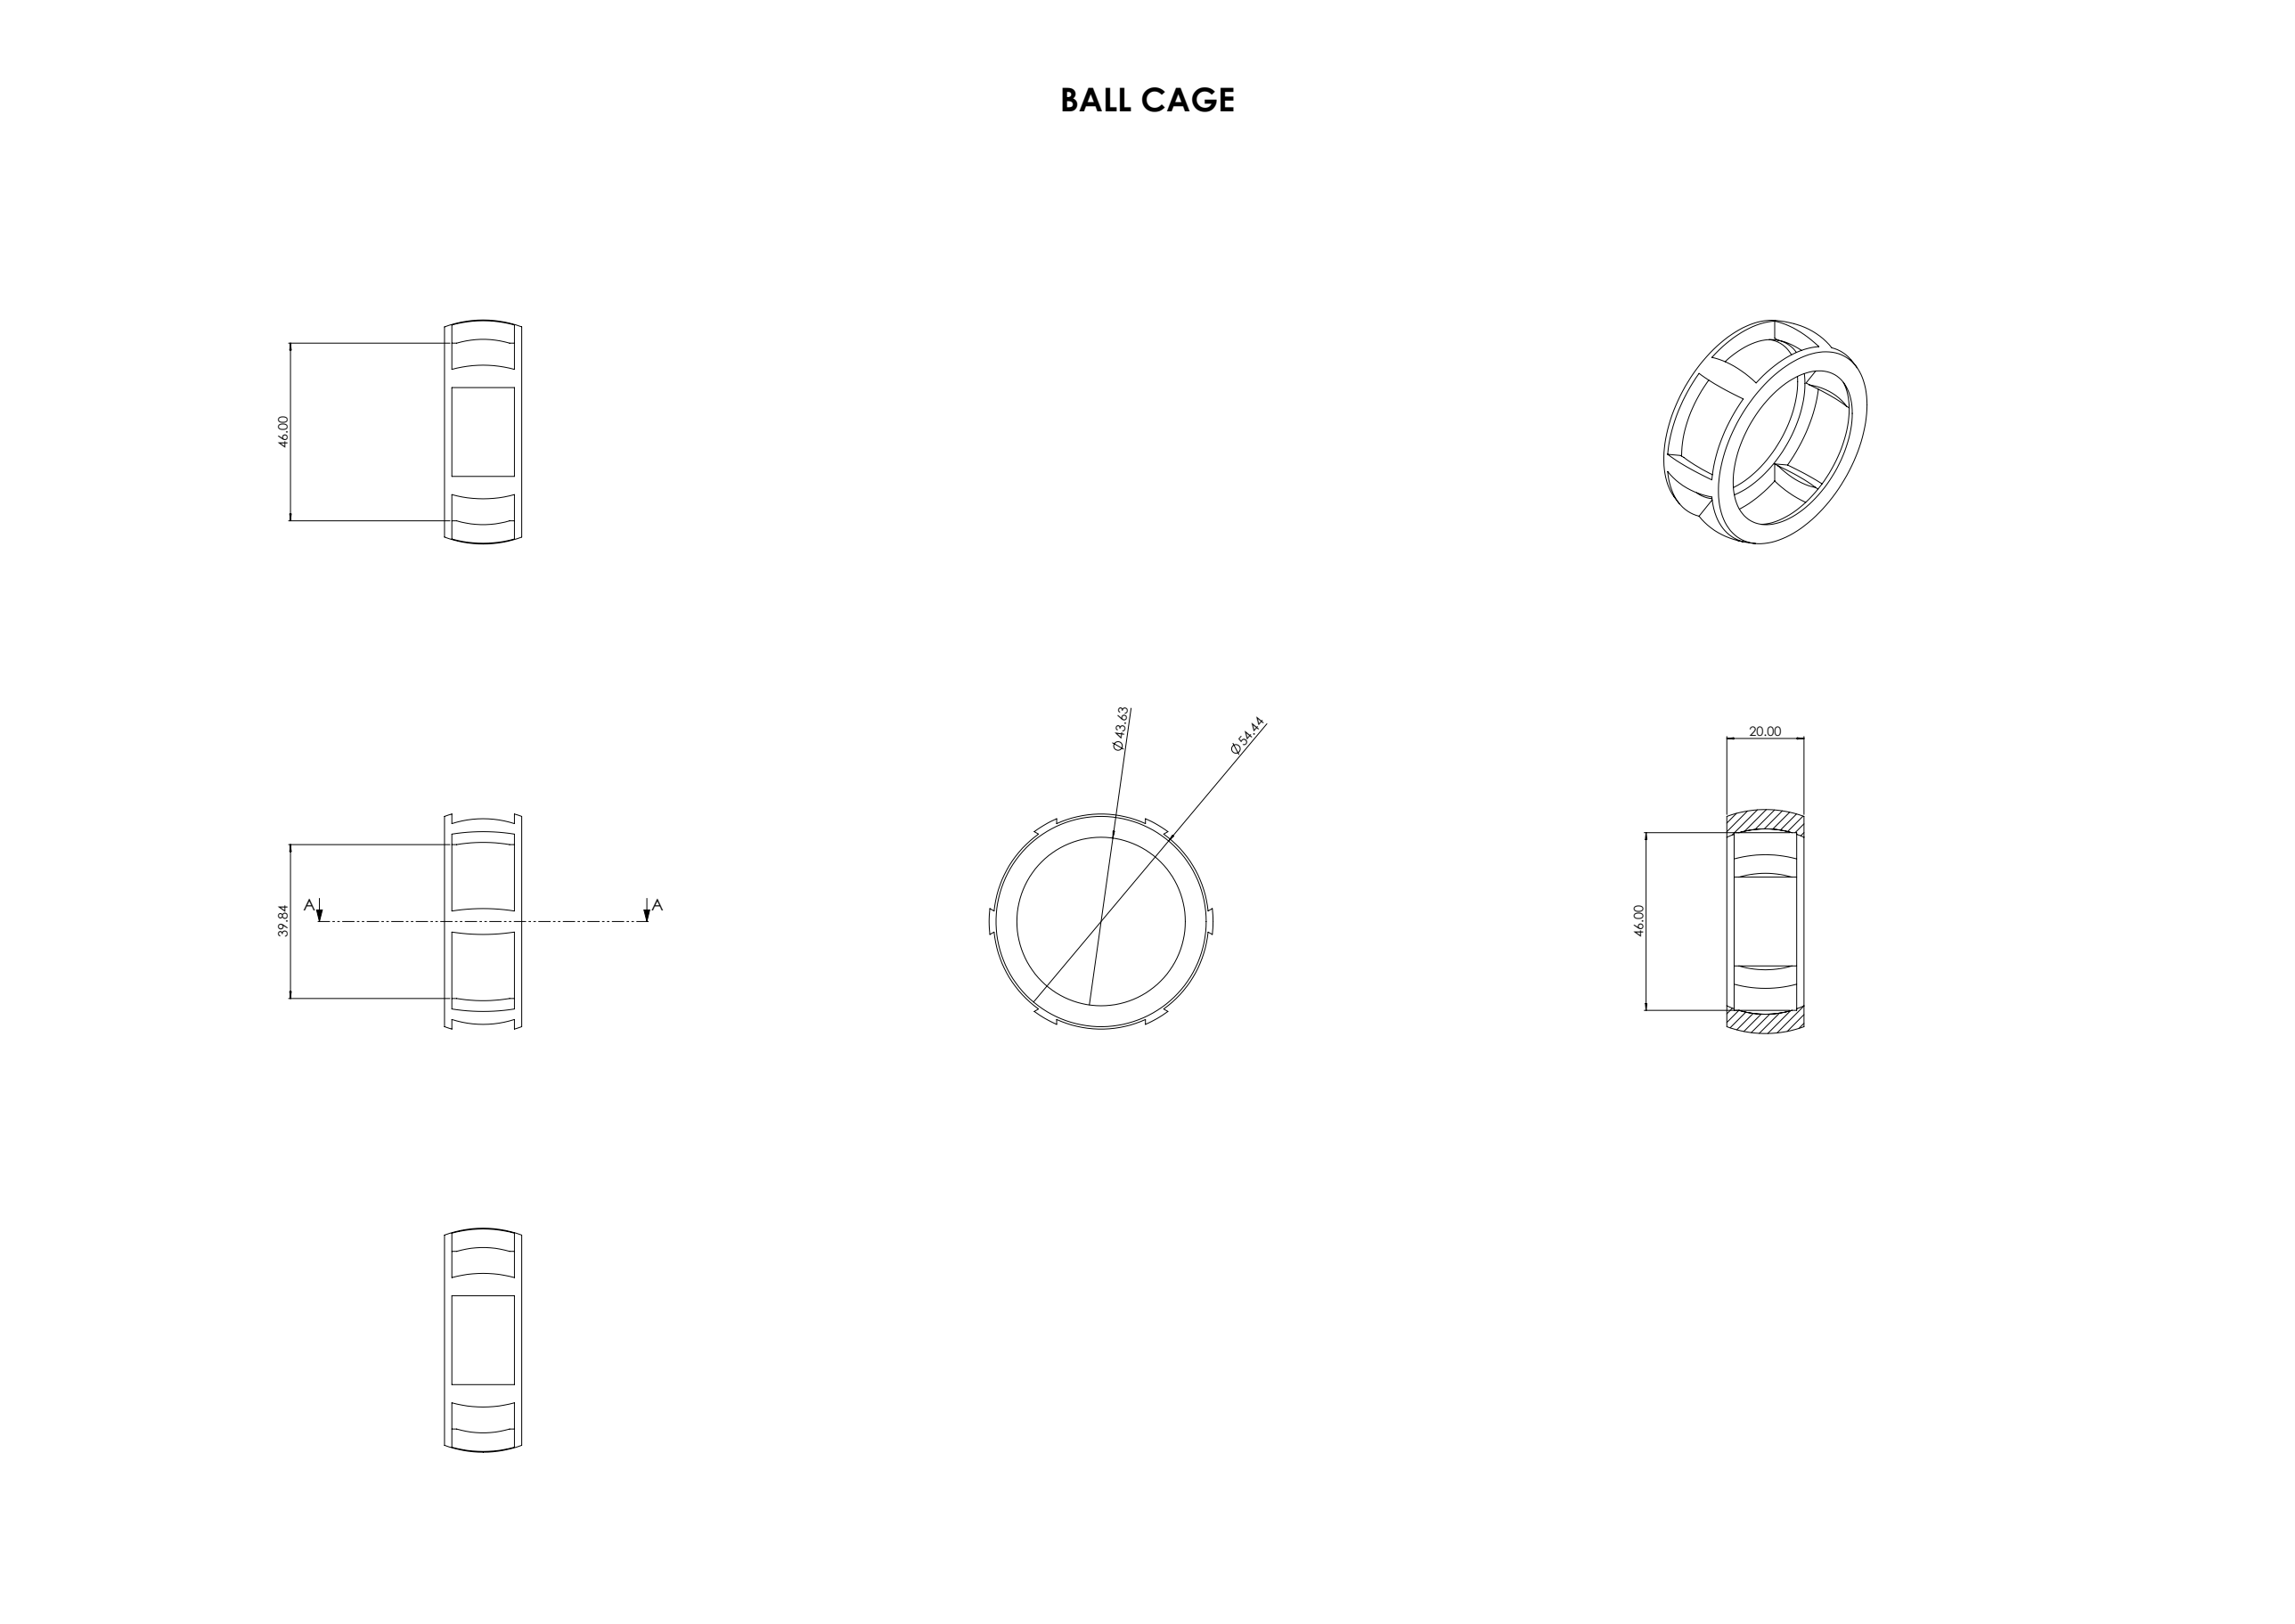
ISO-10303-21;
HEADER;
/* Generated by software containing ST-Developer
 * from STEP Tools, Inc. (www.steptools.com) 
 */

FILE_DESCRIPTION(
/* description */ (''),
/* implementation_level */ '2;1');

FILE_NAME(
/* name */ '05_Ball_Cage.step',
/* time_stamp */ '2026-10-11T12:57:03-07:00',
/* author */ (''),
/* organization */ (''),
/* preprocessor_version */ 'ST-DEVELOPER v20.2',
/* originating_system */ 'Autodesk Translation Framework v15.15.0.0',
/* authorisation */ '');

FILE_SCHEMA (('AUTOMOTIVE_DESIGN { 1 0 10303 214 3 1 1 }'));
ENDSEC;

DATA;
#10=MECHANICAL_DESIGN_GEOMETRIC_PRESENTATION_REPRESENTATION('',(#260),#90374);
#226=SHAPE_REPRESENTATION_RELATIONSHIP('SRR','None',#90445,#243);
#243=ADVANCED_BREP_SHAPE_REPRESENTATION('',(#277),#90361);
#260=STYLED_ITEM('',(#90701),#277);
#277=MANIFOLD_SOLID_BREP('Body1',#40349);
#557=SPHERICAL_SURFACE('',#43737,24.);
#558=SPHERICAL_SURFACE('',#43740,24.);
#559=SPHERICAL_SURFACE('',#43742,24.);
#560=SPHERICAL_SURFACE('',#43747,24.);
#561=SPHERICAL_SURFACE('',#43754,24.);
#562=SPHERICAL_SURFACE('',#43761,24.);
#563=SPHERICAL_SURFACE('',#43769,24.);
#564=SPHERICAL_SURFACE('',#43785,24.);
#565=SPHERICAL_SURFACE('',#43789,29.);
#1053=FACE_BOUND('',#6193,.T.);
#1054=FACE_BOUND('',#6196,.T.);
#1055=FACE_BOUND('',#6213,.T.);
#1056=FACE_BOUND('',#6215,.T.);
#1057=FACE_BOUND('',#6217,.T.);
#1058=FACE_BOUND('',#6219,.T.);
#1059=FACE_BOUND('',#6221,.T.);
#1060=FACE_BOUND('',#6222,.T.);
#1061=FACE_BOUND('',#6223,.T.);
#1062=FACE_BOUND('',#6224,.T.);
#1063=FACE_BOUND('',#6225,.T.);
#1064=FACE_BOUND('',#6226,.T.);
#1065=FACE_BOUND('',#6227,.T.);
#1420=PLANE('',#43720);
#1421=PLANE('',#43723);
#1422=PLANE('',#43726);
#1423=PLANE('',#43734);
#1424=PLANE('',#43744);
#1425=PLANE('',#43749);
#1426=PLANE('',#43751);
#1427=PLANE('',#43756);
#1428=PLANE('',#43758);
#1429=PLANE('',#43764);
#1430=PLANE('',#43766);
#1431=PLANE('',#43771);
#1432=PLANE('',#43773);
#1433=PLANE('',#43775);
#1434=PLANE('',#43782);
#1435=PLANE('',#43786);
#3780=FACE_OUTER_BOUND('',#6190,.T.);
#3781=FACE_OUTER_BOUND('',#6191,.T.);
#3782=FACE_OUTER_BOUND('',#6192,.T.);
#3783=FACE_OUTER_BOUND('',#6194,.T.);
#3784=FACE_OUTER_BOUND('',#6195,.T.);
#3785=FACE_OUTER_BOUND('',#6197,.T.);
#3786=FACE_OUTER_BOUND('',#6198,.T.);
#3787=FACE_OUTER_BOUND('',#6199,.T.);
#3788=FACE_OUTER_BOUND('',#6200,.T.);
#3789=FACE_OUTER_BOUND('',#6201,.T.);
#3790=FACE_OUTER_BOUND('',#6202,.T.);
#3791=FACE_OUTER_BOUND('',#6203,.T.);
#3792=FACE_OUTER_BOUND('',#6204,.T.);
#3793=FACE_OUTER_BOUND('',#6205,.T.);
#3794=FACE_OUTER_BOUND('',#6206,.T.);
#3795=FACE_OUTER_BOUND('',#6207,.T.);
#3796=FACE_OUTER_BOUND('',#6208,.T.);
#3797=FACE_OUTER_BOUND('',#6209,.T.);
#3798=FACE_OUTER_BOUND('',#6210,.T.);
#3799=FACE_OUTER_BOUND('',#6211,.T.);
#3800=FACE_OUTER_BOUND('',#6212,.T.);
#3801=FACE_OUTER_BOUND('',#6214,.T.);
#3802=FACE_OUTER_BOUND('',#6216,.T.);
#3803=FACE_OUTER_BOUND('',#6218,.T.);
#3804=FACE_OUTER_BOUND('',#6220,.T.);
#6190=EDGE_LOOP('',(#33099,#33100,#33101,#33102,#33103,#33104));
#6191=EDGE_LOOP('',(#33105,#33106,#33107,#33108,#33109,#33110));
#6192=EDGE_LOOP('',(#33111,#33112,#33113,#33114,#33115,#33116,#33117,#33118,
#33119,#33120,#33121,#33122,#33123,#33124,#33125,#33126,#33127,#33128));
#6193=EDGE_LOOP('',(#33129));
#6194=EDGE_LOOP('',(#33130,#33131,#33132,#33133,#33134,#33135));
#6195=EDGE_LOOP('',(#33136));
#6196=EDGE_LOOP('',(#33137));
#6197=EDGE_LOOP('',(#33138,#33139,#33140,#33141));
#6198=EDGE_LOOP('',(#33142,#33143));
#6199=EDGE_LOOP('',(#33144,#33145,#33146,#33147,#33148,#33149));
#6200=EDGE_LOOP('',(#33150,#33151));
#6201=EDGE_LOOP('',(#33152,#33153,#33154,#33155,#33156,#33157));
#6202=EDGE_LOOP('',(#33158,#33159,#33160,#33161,#33162,#33163));
#6203=EDGE_LOOP('',(#33164,#33165));
#6204=EDGE_LOOP('',(#33166,#33167,#33168,#33169,#33170,#33171));
#6205=EDGE_LOOP('',(#33172,#33173,#33174,#33175,#33176,#33177));
#6206=EDGE_LOOP('',(#33178,#33179,#33180,#33181));
#6207=EDGE_LOOP('',(#33182,#33183,#33184,#33185,#33186,#33187));
#6208=EDGE_LOOP('',(#33188,#33189,#33190,#33191,#33192,#33193));
#6209=EDGE_LOOP('',(#33194,#33195));
#6210=EDGE_LOOP('',(#33196,#33197,#33198,#33199,#33200,#33201));
#6211=EDGE_LOOP('',(#33202,#33203,#33204,#33205,#33206,#33207));
#6212=EDGE_LOOP('',(#33208,#33209,#33210,#33211,#33212,#33213,#33214,#33215,
#33216,#33217,#33218,#33219,#33220,#33221,#33222,#33223,#33224,#33225));
#6213=EDGE_LOOP('',(#33226));
#6214=EDGE_LOOP('',(#33227));
#6215=EDGE_LOOP('',(#33228));
#6216=EDGE_LOOP('',(#33229));
#6217=EDGE_LOOP('',(#33230));
#6218=EDGE_LOOP('',(#33231,#33232));
#6219=EDGE_LOOP('',(#33233));
#6220=EDGE_LOOP('',(#33234,#33235,#33236,#33237,#33238,#33239));
#6221=EDGE_LOOP('',(#33240,#33241,#33242,#33243));
#6222=EDGE_LOOP('',(#33244,#33245,#33246,#33247));
#6223=EDGE_LOOP('',(#33248,#33249,#33250,#33251));
#6224=EDGE_LOOP('',(#33252,#33253,#33254,#33255));
#6225=EDGE_LOOP('',(#33256,#33257,#33258,#33259));
#6226=EDGE_LOOP('',(#33260,#33261,#33262,#33263));
#6227=EDGE_LOOP('',(#33264));
#8631=CIRCLE('',#43721,26.6223590239483);
#8632=CIRCLE('',#43722,21.0653744329409);
#8633=CIRCLE('',#43724,26.6223590239483);
#8634=CIRCLE('',#43725,21.0653744329409);
#8635=CIRCLE('',#43727,27.8458255399261);
#8636=CIRCLE('',#43728,27.8458255399261);
#8637=CIRCLE('',#43729,27.8458255399261);
#8638=CIRCLE('',#43730,27.8458255399261);
#8639=CIRCLE('',#43731,27.8458255399261);
#8640=CIRCLE('',#43732,27.8458255399261);
#8641=CIRCLE('',#43733,22.5918126762773);
#8642=CIRCLE('',#43735,21.0653744329409);
#8643=CIRCLE('',#43736,26.6223590239483);
#8644=CIRCLE('',#43738,22.5918126762773);
#8645=CIRCLE('',#43739,21.8174242292714);
#8646=CIRCLE('',#43741,24.);
#8647=CIRCLE('',#43743,21.0653744329409);
#8648=CIRCLE('',#43745,26.6223590239483);
#8649=CIRCLE('',#43746,21.0653744329409);
#8650=CIRCLE('',#43748,21.0653744329409);
#8651=CIRCLE('',#43750,26.6223590239483);
#8652=CIRCLE('',#43752,26.6223590239483);
#8653=CIRCLE('',#43753,21.0653744329409);
#8654=CIRCLE('',#43755,21.0653744329409);
#8655=CIRCLE('',#43757,26.6223590239483);
#8656=CIRCLE('',#43759,26.6223590239483);
#8657=CIRCLE('',#43760,21.0653744329409);
#8658=CIRCLE('',#43762,24.);
#8659=CIRCLE('',#43763,21.0653744329409);
#8660=CIRCLE('',#43765,26.6223590239483);
#8661=CIRCLE('',#43767,26.6223590239483);
#8662=CIRCLE('',#43768,21.0653744329409);
#8663=CIRCLE('',#43770,21.0653744329409);
#8664=CIRCLE('',#43772,26.6223590239483);
#8665=CIRCLE('',#43774,26.6223590239483);
#8666=CIRCLE('',#43776,27.8458255399261);
#8667=CIRCLE('',#43777,27.8458255399261);
#8668=CIRCLE('',#43778,27.8458255399261);
#8669=CIRCLE('',#43779,27.8458255399261);
#8670=CIRCLE('',#43780,27.8458255399261);
#8671=CIRCLE('',#43781,27.8458255399261);
#8672=CIRCLE('',#43783,27.2213151776324);
#8673=CIRCLE('',#43784,21.8174242292714);
#8674=CIRCLE('',#43787,27.2213151776324);
#8675=CIRCLE('',#43788,27.2213151776324);
#8676=CIRCLE('',#43790,29.);
#8677=CIRCLE('',#43791,29.);
#11805=LINE('',#81064,#14299);
#11806=LINE('',#81066,#14300);
#11807=LINE('',#81070,#14301);
#11808=LINE('',#81071,#14302);
#11809=LINE('',#81077,#14303);
#11810=LINE('',#81079,#14304);
#11811=LINE('',#81083,#14305);
#11812=LINE('',#81084,#14306);
#11813=LINE('',#81087,#14307);
#11814=LINE('',#81091,#14308);
#11815=LINE('',#81093,#14309);
#11816=LINE('',#81097,#14310);
#11817=LINE('',#81099,#14311);
#11818=LINE('',#81103,#14312);
#11819=LINE('',#81105,#14313);
#11820=LINE('',#81109,#14314);
#11821=LINE('',#81111,#14315);
#11822=LINE('',#81114,#14316);
#11823=LINE('',#81121,#14317);
#11824=LINE('',#81135,#14318);
#11825=LINE('',#81139,#14319);
#11826=LINE('',#81141,#14320);
#11827=LINE('',#81147,#14321);
#11828=LINE('',#81151,#14322);
#11829=LINE('',#81155,#14323);
#11830=LINE('',#81157,#14324);
#11831=LINE('',#81163,#14325);
#11832=LINE('',#81167,#14326);
#11833=LINE('',#81171,#14327);
#11834=LINE('',#81173,#14328);
#11835=LINE('',#81181,#14329);
#11836=LINE('',#81185,#14330);
#11837=LINE('',#81189,#14331);
#11838=LINE('',#81191,#14332);
#11839=LINE('',#81197,#14333);
#11840=LINE('',#81202,#14334);
#14299=VECTOR('',#53087,10.);
#14300=VECTOR('',#53088,10.);
#14301=VECTOR('',#53091,10.);
#14302=VECTOR('',#53092,10.);
#14303=VECTOR('',#53097,10.);
#14304=VECTOR('',#53098,10.);
#14305=VECTOR('',#53101,10.);
#14306=VECTOR('',#53102,10.);
#14307=VECTOR('',#53105,10.);
#14308=VECTOR('',#53108,10.);
#14309=VECTOR('',#53109,10.);
#14310=VECTOR('',#53112,10.);
#14311=VECTOR('',#53113,10.);
#14312=VECTOR('',#53116,10.);
#14313=VECTOR('',#53117,10.);
#14314=VECTOR('',#53120,10.);
#14315=VECTOR('',#53121,10.);
#14316=VECTOR('',#53124,10.);
#14317=VECTOR('',#53133,10.);
#14318=VECTOR('',#53152,10.);
#14319=VECTOR('',#53155,10.);
#14320=VECTOR('',#53156,10.);
#14321=VECTOR('',#53165,10.);
#14322=VECTOR('',#53170,10.);
#14323=VECTOR('',#53173,10.);
#14324=VECTOR('',#53174,10.);
#14325=VECTOR('',#53183,10.);
#14326=VECTOR('',#53188,10.);
#14327=VECTOR('',#53191,10.);
#14328=VECTOR('',#53192,10.);
#14329=VECTOR('',#53203,10.);
#14330=VECTOR('',#53208,10.);
#14331=VECTOR('',#53211,10.);
#14332=VECTOR('',#53212,10.);
#14333=VECTOR('',#53221,10.);
#14334=VECTOR('',#53228,10.);
#17713=VERTEX_POINT('',#81060);
#17714=VERTEX_POINT('',#81061);
#17715=VERTEX_POINT('',#81063);
#17716=VERTEX_POINT('',#81065);
#17717=VERTEX_POINT('',#81067);
#17718=VERTEX_POINT('',#81069);
#17719=VERTEX_POINT('',#81073);
#17720=VERTEX_POINT('',#81074);
#17721=VERTEX_POINT('',#81076);
#17722=VERTEX_POINT('',#81078);
#17723=VERTEX_POINT('',#81080);
#17724=VERTEX_POINT('',#81082);
#17725=VERTEX_POINT('',#81086);
#17726=VERTEX_POINT('',#81088);
#17727=VERTEX_POINT('',#81090);
#17728=VERTEX_POINT('',#81092);
#17729=VERTEX_POINT('',#81094);
#17730=VERTEX_POINT('',#81096);
#17731=VERTEX_POINT('',#81098);
#17732=VERTEX_POINT('',#81100);
#17733=VERTEX_POINT('',#81102);
#17734=VERTEX_POINT('',#81104);
#17735=VERTEX_POINT('',#81106);
#17736=VERTEX_POINT('',#81108);
#17737=VERTEX_POINT('',#81110);
#17738=VERTEX_POINT('',#81112);
#17739=VERTEX_POINT('',#81116);
#17740=VERTEX_POINT('',#81120);
#17741=VERTEX_POINT('',#81124);
#17742=VERTEX_POINT('',#81126);
#17743=VERTEX_POINT('',#81129);
#17744=VERTEX_POINT('',#81134);
#17745=VERTEX_POINT('',#81136);
#17746=VERTEX_POINT('',#81138);
#17747=VERTEX_POINT('',#81140);
#17748=VERTEX_POINT('',#81146);
#17749=VERTEX_POINT('',#81150);
#17750=VERTEX_POINT('',#81152);
#17751=VERTEX_POINT('',#81154);
#17752=VERTEX_POINT('',#81156);
#17753=VERTEX_POINT('',#81162);
#17754=VERTEX_POINT('',#81166);
#17755=VERTEX_POINT('',#81168);
#17756=VERTEX_POINT('',#81170);
#17757=VERTEX_POINT('',#81172);
#17758=VERTEX_POINT('',#81176);
#17759=VERTEX_POINT('',#81180);
#17760=VERTEX_POINT('',#81184);
#17761=VERTEX_POINT('',#81186);
#17762=VERTEX_POINT('',#81188);
#17763=VERTEX_POINT('',#81190);
#17764=VERTEX_POINT('',#81196);
#17765=VERTEX_POINT('',#81200);
#17766=VERTEX_POINT('',#81211);
#17767=VERTEX_POINT('',#81213);
#17768=VERTEX_POINT('',#81217);
#17769=VERTEX_POINT('',#81218);
#17770=VERTEX_POINT('',#81222);
#17771=VERTEX_POINT('',#81224);
#23061=EDGE_CURVE('',#17713,#17714,#8631,.T.);
#23062=EDGE_CURVE('',#17715,#17713,#11805,.T.);
#23063=EDGE_CURVE('',#17716,#17715,#11806,.T.);
#23064=EDGE_CURVE('',#17717,#17716,#8632,.T.);
#23065=EDGE_CURVE('',#17718,#17717,#11807,.T.);
#23066=EDGE_CURVE('',#17714,#17718,#11808,.T.);
#23067=EDGE_CURVE('',#17719,#17720,#8633,.T.);
#23068=EDGE_CURVE('',#17721,#17719,#11809,.T.);
#23069=EDGE_CURVE('',#17722,#17721,#11810,.T.);
#23070=EDGE_CURVE('',#17723,#17722,#8634,.T.);
#23071=EDGE_CURVE('',#17724,#17723,#11811,.T.);
#23072=EDGE_CURVE('',#17720,#17724,#11812,.T.);
#23073=EDGE_CURVE('',#17724,#17725,#11813,.T.);
#23074=EDGE_CURVE('',#17726,#17725,#8635,.T.);
#23075=EDGE_CURVE('',#17726,#17727,#11814,.T.);
#23076=EDGE_CURVE('',#17727,#17728,#11815,.T.);
#23077=EDGE_CURVE('',#17729,#17728,#8636,.T.);
#23078=EDGE_CURVE('',#17729,#17730,#11816,.T.);
#23079=EDGE_CURVE('',#17730,#17731,#11817,.T.);
#23080=EDGE_CURVE('',#17732,#17731,#8637,.T.);
#23081=EDGE_CURVE('',#17732,#17733,#11818,.T.);
#23082=EDGE_CURVE('',#17733,#17734,#11819,.T.);
#23083=EDGE_CURVE('',#17735,#17734,#8638,.T.);
#23084=EDGE_CURVE('',#17735,#17736,#11820,.T.);
#23085=EDGE_CURVE('',#17736,#17737,#11821,.T.);
#23086=EDGE_CURVE('',#17738,#17737,#8639,.T.);
#23087=EDGE_CURVE('',#17738,#17715,#11822,.T.);
#23088=EDGE_CURVE('',#17720,#17713,#8640,.T.);
#23089=EDGE_CURVE('',#17739,#17739,#8641,.T.);
#23090=EDGE_CURVE('',#17722,#17723,#8642,.T.);
#23091=EDGE_CURVE('',#17740,#17721,#11823,.T.);
#23092=EDGE_CURVE('',#17725,#17740,#8643,.T.);
#23093=EDGE_CURVE('',#17741,#17741,#8644,.T.);
#23094=EDGE_CURVE('',#17742,#17742,#8645,.T.);
#23095=EDGE_CURVE('',#17722,#17743,#8646,.T.);
#23096=EDGE_CURVE('',#17716,#17717,#8647,.T.);
#23097=EDGE_CURVE('',#17727,#17744,#11824,.T.);
#23098=EDGE_CURVE('',#17745,#17726,#8648,.T.);
#23099=EDGE_CURVE('',#17746,#17745,#11825,.T.);
#23100=EDGE_CURVE('',#17747,#17746,#11826,.T.);
#23101=EDGE_CURVE('',#17744,#17747,#8649,.T.);
#23102=EDGE_CURVE('',#17747,#17744,#8650,.T.);
#23103=EDGE_CURVE('',#17748,#17746,#11827,.T.);
#23104=EDGE_CURVE('',#17728,#17748,#8651,.T.);
#23105=EDGE_CURVE('',#17730,#17749,#11828,.T.);
#23106=EDGE_CURVE('',#17750,#17729,#8652,.T.);
#23107=EDGE_CURVE('',#17751,#17750,#11829,.T.);
#23108=EDGE_CURVE('',#17752,#17751,#11830,.T.);
#23109=EDGE_CURVE('',#17749,#17752,#8653,.T.);
#23110=EDGE_CURVE('',#17752,#17749,#8654,.T.);
#23111=EDGE_CURVE('',#17753,#17751,#11831,.T.);
#23112=EDGE_CURVE('',#17731,#17753,#8655,.T.);
#23113=EDGE_CURVE('',#17733,#17754,#11832,.T.);
#23114=EDGE_CURVE('',#17755,#17732,#8656,.T.);
#23115=EDGE_CURVE('',#17756,#17755,#11833,.T.);
#23116=EDGE_CURVE('',#17757,#17756,#11834,.T.);
#23117=EDGE_CURVE('',#17754,#17757,#8657,.T.);
#23118=EDGE_CURVE('',#17758,#17757,#8658,.T.);
#23119=EDGE_CURVE('',#17757,#17754,#8659,.T.);
#23120=EDGE_CURVE('',#17759,#17756,#11835,.T.);
#23121=EDGE_CURVE('',#17734,#17759,#8660,.T.);
#23122=EDGE_CURVE('',#17736,#17760,#11836,.T.);
#23123=EDGE_CURVE('',#17761,#17735,#8661,.T.);
#23124=EDGE_CURVE('',#17762,#17761,#11837,.T.);
#23125=EDGE_CURVE('',#17763,#17762,#11838,.T.);
#23126=EDGE_CURVE('',#17760,#17763,#8662,.T.);
#23127=EDGE_CURVE('',#17763,#17760,#8663,.T.);
#23128=EDGE_CURVE('',#17764,#17762,#11839,.T.);
#23129=EDGE_CURVE('',#17737,#17764,#8664,.T.);
#23130=EDGE_CURVE('',#17765,#17738,#8665,.T.);
#23131=EDGE_CURVE('',#17718,#17765,#11840,.T.);
#23132=EDGE_CURVE('',#17714,#17719,#8666,.T.);
#23133=EDGE_CURVE('',#17764,#17765,#8667,.T.);
#23134=EDGE_CURVE('',#17759,#17761,#8668,.T.);
#23135=EDGE_CURVE('',#17753,#17755,#8669,.T.);
#23136=EDGE_CURVE('',#17748,#17750,#8670,.T.);
#23137=EDGE_CURVE('',#17740,#17745,#8671,.T.);
#23138=EDGE_CURVE('',#17766,#17766,#8672,.T.);
#23139=EDGE_CURVE('',#17767,#17767,#8673,.T.);
#23140=EDGE_CURVE('',#17768,#17769,#8674,.T.);
#23141=EDGE_CURVE('',#17769,#17768,#8675,.T.);
#23142=EDGE_CURVE('',#17770,#17769,#8676,.T.);
#23143=EDGE_CURVE('',#17768,#17771,#8677,.T.);
#33099=ORIENTED_EDGE('',*,*,#23061,.F.);
#33100=ORIENTED_EDGE('',*,*,#23062,.F.);
#33101=ORIENTED_EDGE('',*,*,#23063,.F.);
#33102=ORIENTED_EDGE('',*,*,#23064,.F.);
#33103=ORIENTED_EDGE('',*,*,#23065,.F.);
#33104=ORIENTED_EDGE('',*,*,#23066,.F.);
#33105=ORIENTED_EDGE('',*,*,#23067,.F.);
#33106=ORIENTED_EDGE('',*,*,#23068,.F.);
#33107=ORIENTED_EDGE('',*,*,#23069,.F.);
#33108=ORIENTED_EDGE('',*,*,#23070,.F.);
#33109=ORIENTED_EDGE('',*,*,#23071,.F.);
#33110=ORIENTED_EDGE('',*,*,#23072,.F.);
#33111=ORIENTED_EDGE('',*,*,#23073,.T.);
#33112=ORIENTED_EDGE('',*,*,#23074,.F.);
#33113=ORIENTED_EDGE('',*,*,#23075,.T.);
#33114=ORIENTED_EDGE('',*,*,#23076,.T.);
#33115=ORIENTED_EDGE('',*,*,#23077,.F.);
#33116=ORIENTED_EDGE('',*,*,#23078,.T.);
#33117=ORIENTED_EDGE('',*,*,#23079,.T.);
#33118=ORIENTED_EDGE('',*,*,#23080,.F.);
#33119=ORIENTED_EDGE('',*,*,#23081,.T.);
#33120=ORIENTED_EDGE('',*,*,#23082,.T.);
#33121=ORIENTED_EDGE('',*,*,#23083,.F.);
#33122=ORIENTED_EDGE('',*,*,#23084,.T.);
#33123=ORIENTED_EDGE('',*,*,#23085,.T.);
#33124=ORIENTED_EDGE('',*,*,#23086,.F.);
#33125=ORIENTED_EDGE('',*,*,#23087,.T.);
#33126=ORIENTED_EDGE('',*,*,#23062,.T.);
#33127=ORIENTED_EDGE('',*,*,#23088,.F.);
#33128=ORIENTED_EDGE('',*,*,#23072,.T.);
#33129=ORIENTED_EDGE('',*,*,#23089,.F.);
#33130=ORIENTED_EDGE('',*,*,#23071,.T.);
#33131=ORIENTED_EDGE('',*,*,#23090,.F.);
#33132=ORIENTED_EDGE('',*,*,#23069,.T.);
#33133=ORIENTED_EDGE('',*,*,#23091,.F.);
#33134=ORIENTED_EDGE('',*,*,#23092,.F.);
#33135=ORIENTED_EDGE('',*,*,#23073,.F.);
#33136=ORIENTED_EDGE('',*,*,#23093,.T.);
#33137=ORIENTED_EDGE('',*,*,#23094,.F.);
#33138=ORIENTED_EDGE('',*,*,#23070,.T.);
#33139=ORIENTED_EDGE('',*,*,#23095,.T.);
#33140=ORIENTED_EDGE('',*,*,#23095,.F.);
#33141=ORIENTED_EDGE('',*,*,#23090,.T.);
#33142=ORIENTED_EDGE('',*,*,#23064,.T.);
#33143=ORIENTED_EDGE('',*,*,#23096,.T.);
#33144=ORIENTED_EDGE('',*,*,#23097,.F.);
#33145=ORIENTED_EDGE('',*,*,#23075,.F.);
#33146=ORIENTED_EDGE('',*,*,#23098,.F.);
#33147=ORIENTED_EDGE('',*,*,#23099,.F.);
#33148=ORIENTED_EDGE('',*,*,#23100,.F.);
#33149=ORIENTED_EDGE('',*,*,#23101,.F.);
#33150=ORIENTED_EDGE('',*,*,#23101,.T.);
#33151=ORIENTED_EDGE('',*,*,#23102,.T.);
#33152=ORIENTED_EDGE('',*,*,#23097,.T.);
#33153=ORIENTED_EDGE('',*,*,#23102,.F.);
#33154=ORIENTED_EDGE('',*,*,#23100,.T.);
#33155=ORIENTED_EDGE('',*,*,#23103,.F.);
#33156=ORIENTED_EDGE('',*,*,#23104,.F.);
#33157=ORIENTED_EDGE('',*,*,#23076,.F.);
#33158=ORIENTED_EDGE('',*,*,#23105,.F.);
#33159=ORIENTED_EDGE('',*,*,#23078,.F.);
#33160=ORIENTED_EDGE('',*,*,#23106,.F.);
#33161=ORIENTED_EDGE('',*,*,#23107,.F.);
#33162=ORIENTED_EDGE('',*,*,#23108,.F.);
#33163=ORIENTED_EDGE('',*,*,#23109,.F.);
#33164=ORIENTED_EDGE('',*,*,#23109,.T.);
#33165=ORIENTED_EDGE('',*,*,#23110,.T.);
#33166=ORIENTED_EDGE('',*,*,#23105,.T.);
#33167=ORIENTED_EDGE('',*,*,#23110,.F.);
#33168=ORIENTED_EDGE('',*,*,#23108,.T.);
#33169=ORIENTED_EDGE('',*,*,#23111,.F.);
#33170=ORIENTED_EDGE('',*,*,#23112,.F.);
#33171=ORIENTED_EDGE('',*,*,#23079,.F.);
#33172=ORIENTED_EDGE('',*,*,#23113,.F.);
#33173=ORIENTED_EDGE('',*,*,#23081,.F.);
#33174=ORIENTED_EDGE('',*,*,#23114,.F.);
#33175=ORIENTED_EDGE('',*,*,#23115,.F.);
#33176=ORIENTED_EDGE('',*,*,#23116,.F.);
#33177=ORIENTED_EDGE('',*,*,#23117,.F.);
#33178=ORIENTED_EDGE('',*,*,#23117,.T.);
#33179=ORIENTED_EDGE('',*,*,#23118,.F.);
#33180=ORIENTED_EDGE('',*,*,#23118,.T.);
#33181=ORIENTED_EDGE('',*,*,#23119,.T.);
#33182=ORIENTED_EDGE('',*,*,#23113,.T.);
#33183=ORIENTED_EDGE('',*,*,#23119,.F.);
#33184=ORIENTED_EDGE('',*,*,#23116,.T.);
#33185=ORIENTED_EDGE('',*,*,#23120,.F.);
#33186=ORIENTED_EDGE('',*,*,#23121,.F.);
#33187=ORIENTED_EDGE('',*,*,#23082,.F.);
#33188=ORIENTED_EDGE('',*,*,#23122,.F.);
#33189=ORIENTED_EDGE('',*,*,#23084,.F.);
#33190=ORIENTED_EDGE('',*,*,#23123,.F.);
#33191=ORIENTED_EDGE('',*,*,#23124,.F.);
#33192=ORIENTED_EDGE('',*,*,#23125,.F.);
#33193=ORIENTED_EDGE('',*,*,#23126,.F.);
#33194=ORIENTED_EDGE('',*,*,#23126,.T.);
#33195=ORIENTED_EDGE('',*,*,#23127,.T.);
#33196=ORIENTED_EDGE('',*,*,#23122,.T.);
#33197=ORIENTED_EDGE('',*,*,#23127,.F.);
#33198=ORIENTED_EDGE('',*,*,#23125,.T.);
#33199=ORIENTED_EDGE('',*,*,#23128,.F.);
#33200=ORIENTED_EDGE('',*,*,#23129,.F.);
#33201=ORIENTED_EDGE('',*,*,#23085,.F.);
#33202=ORIENTED_EDGE('',*,*,#23063,.T.);
#33203=ORIENTED_EDGE('',*,*,#23087,.F.);
#33204=ORIENTED_EDGE('',*,*,#23130,.F.);
#33205=ORIENTED_EDGE('',*,*,#23131,.F.);
#33206=ORIENTED_EDGE('',*,*,#23065,.T.);
#33207=ORIENTED_EDGE('',*,*,#23096,.F.);
#33208=ORIENTED_EDGE('',*,*,#23068,.T.);
#33209=ORIENTED_EDGE('',*,*,#23132,.F.);
#33210=ORIENTED_EDGE('',*,*,#23066,.T.);
#33211=ORIENTED_EDGE('',*,*,#23131,.T.);
#33212=ORIENTED_EDGE('',*,*,#23133,.F.);
#33213=ORIENTED_EDGE('',*,*,#23128,.T.);
#33214=ORIENTED_EDGE('',*,*,#23124,.T.);
#33215=ORIENTED_EDGE('',*,*,#23134,.F.);
#33216=ORIENTED_EDGE('',*,*,#23120,.T.);
#33217=ORIENTED_EDGE('',*,*,#23115,.T.);
#33218=ORIENTED_EDGE('',*,*,#23135,.F.);
#33219=ORIENTED_EDGE('',*,*,#23111,.T.);
#33220=ORIENTED_EDGE('',*,*,#23107,.T.);
#33221=ORIENTED_EDGE('',*,*,#23136,.F.);
#33222=ORIENTED_EDGE('',*,*,#23103,.T.);
#33223=ORIENTED_EDGE('',*,*,#23099,.T.);
#33224=ORIENTED_EDGE('',*,*,#23137,.F.);
#33225=ORIENTED_EDGE('',*,*,#23091,.T.);
#33226=ORIENTED_EDGE('',*,*,#23093,.F.);
#33227=ORIENTED_EDGE('',*,*,#23138,.T.);
#33228=ORIENTED_EDGE('',*,*,#23139,.F.);
#33229=ORIENTED_EDGE('',*,*,#23089,.T.);
#33230=ORIENTED_EDGE('',*,*,#23139,.T.);
#33231=ORIENTED_EDGE('',*,*,#23140,.F.);
#33232=ORIENTED_EDGE('',*,*,#23141,.F.);
#33233=ORIENTED_EDGE('',*,*,#23094,.T.);
#33234=ORIENTED_EDGE('',*,*,#23140,.T.);
#33235=ORIENTED_EDGE('',*,*,#23142,.F.);
#33236=ORIENTED_EDGE('',*,*,#23142,.T.);
#33237=ORIENTED_EDGE('',*,*,#23141,.T.);
#33238=ORIENTED_EDGE('',*,*,#23143,.T.);
#33239=ORIENTED_EDGE('',*,*,#23143,.F.);
#33240=ORIENTED_EDGE('',*,*,#23067,.T.);
#33241=ORIENTED_EDGE('',*,*,#23088,.T.);
#33242=ORIENTED_EDGE('',*,*,#23061,.T.);
#33243=ORIENTED_EDGE('',*,*,#23132,.T.);
#33244=ORIENTED_EDGE('',*,*,#23098,.T.);
#33245=ORIENTED_EDGE('',*,*,#23074,.T.);
#33246=ORIENTED_EDGE('',*,*,#23092,.T.);
#33247=ORIENTED_EDGE('',*,*,#23137,.T.);
#33248=ORIENTED_EDGE('',*,*,#23106,.T.);
#33249=ORIENTED_EDGE('',*,*,#23077,.T.);
#33250=ORIENTED_EDGE('',*,*,#23104,.T.);
#33251=ORIENTED_EDGE('',*,*,#23136,.T.);
#33252=ORIENTED_EDGE('',*,*,#23114,.T.);
#33253=ORIENTED_EDGE('',*,*,#23080,.T.);
#33254=ORIENTED_EDGE('',*,*,#23112,.T.);
#33255=ORIENTED_EDGE('',*,*,#23135,.T.);
#33256=ORIENTED_EDGE('',*,*,#23123,.T.);
#33257=ORIENTED_EDGE('',*,*,#23083,.T.);
#33258=ORIENTED_EDGE('',*,*,#23121,.T.);
#33259=ORIENTED_EDGE('',*,*,#23134,.T.);
#33260=ORIENTED_EDGE('',*,*,#23130,.T.);
#33261=ORIENTED_EDGE('',*,*,#23086,.T.);
#33262=ORIENTED_EDGE('',*,*,#23129,.T.);
#33263=ORIENTED_EDGE('',*,*,#23133,.T.);
#33264=ORIENTED_EDGE('',*,*,#23138,.F.);
#39583=ADVANCED_FACE('',(#3780),#1420,.F.);
#39584=ADVANCED_FACE('',(#3781),#1421,.F.);
#39585=ADVANCED_FACE('',(#3782,#1053),#1422,.F.);
#39586=ADVANCED_FACE('',(#3783),#1423,.F.);
#39587=ADVANCED_FACE('',(#3784,#1054),#557,.F.);
#39588=ADVANCED_FACE('',(#3785),#558,.F.);
#39589=ADVANCED_FACE('',(#3786),#559,.F.);
#39590=ADVANCED_FACE('',(#3787),#1424,.F.);
#39591=ADVANCED_FACE('',(#3788),#560,.F.);
#39592=ADVANCED_FACE('',(#3789),#1425,.F.);
#39593=ADVANCED_FACE('',(#3790),#1426,.F.);
#39594=ADVANCED_FACE('',(#3791),#561,.F.);
#39595=ADVANCED_FACE('',(#3792),#1427,.F.);
#39596=ADVANCED_FACE('',(#3793),#1428,.F.);
#39597=ADVANCED_FACE('',(#3794),#562,.F.);
#39598=ADVANCED_FACE('',(#3795),#1429,.F.);
#39599=ADVANCED_FACE('',(#3796),#1430,.F.);
#39600=ADVANCED_FACE('',(#3797),#563,.F.);
#39601=ADVANCED_FACE('',(#3798),#1431,.F.);
#39602=ADVANCED_FACE('',(#3799),#1432,.F.);
#39603=ADVANCED_FACE('',(#3800,#1055),#1433,.F.);
#39604=ADVANCED_FACE('',(#3801,#1056),#1434,.T.);
#39605=ADVANCED_FACE('',(#3802,#1057),#564,.F.);
#39606=ADVANCED_FACE('',(#3803,#1058),#1435,.T.);
#39607=ADVANCED_FACE('',(#3804,#1059,#1060,#1061,#1062,#1063,#1064,#1065),
#565,.T.);
#40349=CLOSED_SHELL('',(#39583,#39584,#39585,#39586,#39587,#39588,#39589,
#39590,#39591,#39592,#39593,#39594,#39595,#39596,#39597,#39598,#39599,#39600,
#39601,#39602,#39603,#39604,#39605,#39606,#39607));
#43719=AXIS2_PLACEMENT_3D('',#81058,#53081,#53082);
#43720=AXIS2_PLACEMENT_3D('',#81059,#53083,#53084);
#43721=AXIS2_PLACEMENT_3D('',#81062,#53085,#53086);
#43722=AXIS2_PLACEMENT_3D('',#81068,#53089,#53090);
#43723=AXIS2_PLACEMENT_3D('',#81072,#53093,#53094);
#43724=AXIS2_PLACEMENT_3D('',#81075,#53095,#53096);
#43725=AXIS2_PLACEMENT_3D('',#81081,#53099,#53100);
#43726=AXIS2_PLACEMENT_3D('',#81085,#53103,#53104);
#43727=AXIS2_PLACEMENT_3D('',#81089,#53106,#53107);
#43728=AXIS2_PLACEMENT_3D('',#81095,#53110,#53111);
#43729=AXIS2_PLACEMENT_3D('',#81101,#53114,#53115);
#43730=AXIS2_PLACEMENT_3D('',#81107,#53118,#53119);
#43731=AXIS2_PLACEMENT_3D('',#81113,#53122,#53123);
#43732=AXIS2_PLACEMENT_3D('',#81115,#53125,#53126);
#43733=AXIS2_PLACEMENT_3D('',#81117,#53127,#53128);
#43734=AXIS2_PLACEMENT_3D('',#81118,#53129,#53130);
#43735=AXIS2_PLACEMENT_3D('',#81119,#53131,#53132);
#43736=AXIS2_PLACEMENT_3D('',#81122,#53134,#53135);
#43737=AXIS2_PLACEMENT_3D('',#81123,#53136,#53137);
#43738=AXIS2_PLACEMENT_3D('',#81125,#53138,#53139);
#43739=AXIS2_PLACEMENT_3D('',#81127,#53140,#53141);
#43740=AXIS2_PLACEMENT_3D('',#81128,#53142,#53143);
#43741=AXIS2_PLACEMENT_3D('',#81130,#53144,#53145);
#43742=AXIS2_PLACEMENT_3D('',#81131,#53146,#53147);
#43743=AXIS2_PLACEMENT_3D('',#81132,#53148,#53149);
#43744=AXIS2_PLACEMENT_3D('',#81133,#53150,#53151);
#43745=AXIS2_PLACEMENT_3D('',#81137,#53153,#53154);
#43746=AXIS2_PLACEMENT_3D('',#81142,#53157,#53158);
#43747=AXIS2_PLACEMENT_3D('',#81143,#53159,#53160);
#43748=AXIS2_PLACEMENT_3D('',#81144,#53161,#53162);
#43749=AXIS2_PLACEMENT_3D('',#81145,#53163,#53164);
#43750=AXIS2_PLACEMENT_3D('',#81148,#53166,#53167);
#43751=AXIS2_PLACEMENT_3D('',#81149,#53168,#53169);
#43752=AXIS2_PLACEMENT_3D('',#81153,#53171,#53172);
#43753=AXIS2_PLACEMENT_3D('',#81158,#53175,#53176);
#43754=AXIS2_PLACEMENT_3D('',#81159,#53177,#53178);
#43755=AXIS2_PLACEMENT_3D('',#81160,#53179,#53180);
#43756=AXIS2_PLACEMENT_3D('',#81161,#53181,#53182);
#43757=AXIS2_PLACEMENT_3D('',#81164,#53184,#53185);
#43758=AXIS2_PLACEMENT_3D('',#81165,#53186,#53187);
#43759=AXIS2_PLACEMENT_3D('',#81169,#53189,#53190);
#43760=AXIS2_PLACEMENT_3D('',#81174,#53193,#53194);
#43761=AXIS2_PLACEMENT_3D('',#81175,#53195,#53196);
#43762=AXIS2_PLACEMENT_3D('',#81177,#53197,#53198);
#43763=AXIS2_PLACEMENT_3D('',#81178,#53199,#53200);
#43764=AXIS2_PLACEMENT_3D('',#81179,#53201,#53202);
#43765=AXIS2_PLACEMENT_3D('',#81182,#53204,#53205);
#43766=AXIS2_PLACEMENT_3D('',#81183,#53206,#53207);
#43767=AXIS2_PLACEMENT_3D('',#81187,#53209,#53210);
#43768=AXIS2_PLACEMENT_3D('',#81192,#53213,#53214);
#43769=AXIS2_PLACEMENT_3D('',#81193,#53215,#53216);
#43770=AXIS2_PLACEMENT_3D('',#81194,#53217,#53218);
#43771=AXIS2_PLACEMENT_3D('',#81195,#53219,#53220);
#43772=AXIS2_PLACEMENT_3D('',#81198,#53222,#53223);
#43773=AXIS2_PLACEMENT_3D('',#81199,#53224,#53225);
#43774=AXIS2_PLACEMENT_3D('',#81201,#53226,#53227);
#43775=AXIS2_PLACEMENT_3D('',#81203,#53229,#53230);
#43776=AXIS2_PLACEMENT_3D('',#81204,#53231,#53232);
#43777=AXIS2_PLACEMENT_3D('',#81205,#53233,#53234);
#43778=AXIS2_PLACEMENT_3D('',#81206,#53235,#53236);
#43779=AXIS2_PLACEMENT_3D('',#81207,#53237,#53238);
#43780=AXIS2_PLACEMENT_3D('',#81208,#53239,#53240);
#43781=AXIS2_PLACEMENT_3D('',#81209,#53241,#53242);
#43782=AXIS2_PLACEMENT_3D('',#81210,#53243,#53244);
#43783=AXIS2_PLACEMENT_3D('',#81212,#53245,#53246);
#43784=AXIS2_PLACEMENT_3D('',#81214,#53247,#53248);
#43785=AXIS2_PLACEMENT_3D('',#81215,#53249,#53250);
#43786=AXIS2_PLACEMENT_3D('',#81216,#53251,#53252);
#43787=AXIS2_PLACEMENT_3D('',#81219,#53253,#53254);
#43788=AXIS2_PLACEMENT_3D('',#81220,#53255,#53256);
#43789=AXIS2_PLACEMENT_3D('',#81221,#53257,#53258);
#43790=AXIS2_PLACEMENT_3D('',#81223,#53259,#53260);
#43791=AXIS2_PLACEMENT_3D('',#81225,#53261,#53262);
#53081=DIRECTION('axis',(0.,0.,1.));
#53082=DIRECTION('refdir',(1.,0.,0.));
#53083=DIRECTION('center_axis',(0.,0.866025403784439,0.499999999999999));
#53084=DIRECTION('ref_axis',(1.,0.,0.));
#53085=DIRECTION('center_axis',(0.,0.866025403784439,0.499999999999999));
#53086=DIRECTION('ref_axis',(0.,0.499999999999999,-0.866025403784439));
#53087=DIRECTION('',(0.,0.499999999999999,-0.866025403784439));
#53088=DIRECTION('',(1.,0.,0.));
#53089=DIRECTION('center_axis',(0.,-0.866025403784439,-0.499999999999999));
#53090=DIRECTION('ref_axis',(0.,0.499999999999999,-0.866025403784439));
#53091=DIRECTION('',(1.,0.,0.));
#53092=DIRECTION('',(0.,-0.499999999999999,0.866025403784439));
#53093=DIRECTION('center_axis',(0.,-0.866025403784439,-0.499999999999999));
#53094=DIRECTION('ref_axis',(-1.,0.,0.));
#53095=DIRECTION('center_axis',(0.,-0.866025403784439,-0.499999999999999));
#53096=DIRECTION('ref_axis',(0.,-0.499999999999999,0.866025403784439));
#53097=DIRECTION('',(0.,0.499999999999999,-0.866025403784439));
#53098=DIRECTION('',(-1.,0.,0.));
#53099=DIRECTION('center_axis',(0.,0.866025403784439,0.499999999999999));
#53100=DIRECTION('ref_axis',(0.,-0.499999999999999,0.866025403784439));
#53101=DIRECTION('',(-1.,0.,0.));
#53102=DIRECTION('',(0.,-0.499999999999999,0.866025403784439));
#53103=DIRECTION('center_axis',(1.,0.,0.));
#53104=DIRECTION('ref_axis',(0.,1.,0.));
#53105=DIRECTION('',(0.,-0.5,-0.866025403784438));
#53106=DIRECTION('center_axis',(1.,0.,0.));
#53107=DIRECTION('ref_axis',(0.,0.,1.));
#53108=DIRECTION('',(0.,0.5,0.866025403784438));
#53109=DIRECTION('',(0.,-1.,1.22464679914735E-16));
#53110=DIRECTION('center_axis',(1.,0.,0.));
#53111=DIRECTION('ref_axis',(0.,0.,1.));
#53112=DIRECTION('',(0.,1.,-1.22464679914735E-16));
#53113=DIRECTION('',(0.,-0.5,0.866025403784439));
#53114=DIRECTION('center_axis',(1.,0.,0.));
#53115=DIRECTION('ref_axis',(0.,0.,1.));
#53116=DIRECTION('',(0.,0.5,-0.866025403784439));
#53117=DIRECTION('',(0.,0.5,0.866025403784439));
#53118=DIRECTION('center_axis',(1.,0.,0.));
#53119=DIRECTION('ref_axis',(0.,0.,1.));
#53120=DIRECTION('',(0.,-0.5,-0.866025403784439));
#53121=DIRECTION('',(0.,1.,0.));
#53122=DIRECTION('center_axis',(1.,0.,0.));
#53123=DIRECTION('ref_axis',(0.,0.,1.));
#53124=DIRECTION('',(0.,-1.,0.));
#53125=DIRECTION('center_axis',(1.,0.,0.));
#53126=DIRECTION('ref_axis',(0.,0.,1.));
#53127=DIRECTION('center_axis',(-1.,0.,0.));
#53128=DIRECTION('ref_axis',(0.,0.,1.));
#53129=DIRECTION('center_axis',(0.,0.866025403784438,-0.5));
#53130=DIRECTION('ref_axis',(1.,0.,0.));
#53131=DIRECTION('center_axis',(0.,-0.866025403784438,0.5));
#53132=DIRECTION('ref_axis',(0.,-0.5,-0.866025403784438));
#53133=DIRECTION('',(0.,0.5,0.866025403784438));
#53134=DIRECTION('center_axis',(0.,0.866025403784438,-0.5));
#53135=DIRECTION('ref_axis',(0.,-0.5,-0.866025403784438));
#53136=DIRECTION('center_axis',(0.,-9.74610601083004E-20,1.));
#53137=DIRECTION('ref_axis',(-0.999998733308579,-0.00159165990024454,0.));
#53138=DIRECTION('center_axis',(1.,0.,0.));
#53139=DIRECTION('ref_axis',(0.,0.,-1.));
#53140=DIRECTION('center_axis',(1.,0.,0.));
#53141=DIRECTION('ref_axis',(0.,0.,-1.));
#53142=DIRECTION('center_axis',(0.,0.,1.));
#53143=DIRECTION('ref_axis',(1.,0.,0.));
#53144=DIRECTION('center_axis',(1.22464679914735E-16,-1.,0.));
#53145=DIRECTION('ref_axis',(-1.,-1.22464679914735E-16,0.));
#53146=DIRECTION('center_axis',(0.,0.,1.));
#53147=DIRECTION('ref_axis',(1.,0.,0.));
#53148=DIRECTION('center_axis',(0.,0.,1.));
#53149=DIRECTION('ref_axis',(0.,-1.,0.));
#53150=DIRECTION('center_axis',(0.,-0.866025403784438,0.5));
#53151=DIRECTION('ref_axis',(-1.,0.,0.));
#53152=DIRECTION('',(-1.,0.,0.));
#53153=DIRECTION('center_axis',(0.,-0.866025403784438,0.5));
#53154=DIRECTION('ref_axis',(0.,0.5,0.866025403784438));
#53155=DIRECTION('',(0.,-0.5,-0.866025403784438));
#53156=DIRECTION('',(-1.,0.,0.));
#53157=DIRECTION('center_axis',(0.,0.866025403784438,-0.5));
#53158=DIRECTION('ref_axis',(0.,0.5,0.866025403784438));
#53159=DIRECTION('center_axis',(0.,0.,1.));
#53160=DIRECTION('ref_axis',(1.,0.,0.));
#53161=DIRECTION('center_axis',(0.,1.22464679914735E-16,1.));
#53162=DIRECTION('ref_axis',(0.,-1.,1.22464679914735E-16));
#53163=DIRECTION('center_axis',(0.,-1.22464679914735E-16,-1.));
#53164=DIRECTION('ref_axis',(1.,0.,0.));
#53165=DIRECTION('',(0.,1.,-1.22464679914735E-16));
#53166=DIRECTION('center_axis',(0.,-1.22464679914735E-16,-1.));
#53167=DIRECTION('ref_axis',(0.,-1.,1.22464679914735E-16));
#53168=DIRECTION('center_axis',(0.,1.22464679914735E-16,1.));
#53169=DIRECTION('ref_axis',(-1.,0.,0.));
#53170=DIRECTION('',(-1.,0.,0.));
#53171=DIRECTION('center_axis',(0.,1.22464679914735E-16,1.));
#53172=DIRECTION('ref_axis',(0.,1.,-1.22464679914735E-16));
#53173=DIRECTION('',(0.,-1.,1.22464679914735E-16));
#53174=DIRECTION('',(-1.,0.,0.));
#53175=DIRECTION('center_axis',(0.,-1.22464679914735E-16,-1.));
#53176=DIRECTION('ref_axis',(0.,1.,-1.22464679914735E-16));
#53177=DIRECTION('center_axis',(0.,0.,1.));
#53178=DIRECTION('ref_axis',(1.,0.,0.));
#53179=DIRECTION('center_axis',(0.,0.866025403784439,0.5));
#53180=DIRECTION('ref_axis',(0.,-0.5,0.866025403784439));
#53181=DIRECTION('center_axis',(0.,-0.866025403784439,-0.5));
#53182=DIRECTION('ref_axis',(1.,0.,0.));
#53183=DIRECTION('',(0.,0.5,-0.866025403784439));
#53184=DIRECTION('center_axis',(0.,-0.866025403784439,-0.5));
#53185=DIRECTION('ref_axis',(0.,-0.5,0.866025403784439));
#53186=DIRECTION('center_axis',(0.,0.866025403784439,0.5));
#53187=DIRECTION('ref_axis',(-1.,0.,0.));
#53188=DIRECTION('',(-1.,0.,0.));
#53189=DIRECTION('center_axis',(0.,0.866025403784439,0.5));
#53190=DIRECTION('ref_axis',(0.,0.5,-0.866025403784439));
#53191=DIRECTION('',(0.,-0.5,0.866025403784439));
#53192=DIRECTION('',(-1.,0.,0.));
#53193=DIRECTION('center_axis',(0.,-0.866025403784439,-0.5));
#53194=DIRECTION('ref_axis',(0.,0.5,-0.866025403784439));
#53195=DIRECTION('center_axis',(0.,0.,1.));
#53196=DIRECTION('ref_axis',(1.,0.,0.));
#53197=DIRECTION('center_axis',(1.22464679914735E-16,-1.,0.));
#53198=DIRECTION('ref_axis',(-1.,-1.22464679914735E-16,0.));
#53199=DIRECTION('center_axis',(0.,0.866025403784439,-0.5));
#53200=DIRECTION('ref_axis',(0.,0.5,0.866025403784439));
#53201=DIRECTION('center_axis',(0.,-0.866025403784439,0.5));
#53202=DIRECTION('ref_axis',(1.,0.,0.));
#53203=DIRECTION('',(0.,-0.5,-0.866025403784439));
#53204=DIRECTION('center_axis',(0.,-0.866025403784439,0.5));
#53205=DIRECTION('ref_axis',(0.,0.5,0.866025403784438));
#53206=DIRECTION('center_axis',(0.,0.866025403784439,-0.5));
#53207=DIRECTION('ref_axis',(-1.,0.,0.));
#53208=DIRECTION('',(-1.,0.,0.));
#53209=DIRECTION('center_axis',(0.,0.866025403784439,-0.5));
#53210=DIRECTION('ref_axis',(0.,-0.5,-0.866025403784439));
#53211=DIRECTION('',(0.,0.5,0.866025403784439));
#53212=DIRECTION('',(-1.,0.,0.));
#53213=DIRECTION('center_axis',(0.,-0.866025403784439,0.5));
#53214=DIRECTION('ref_axis',(0.,-0.5,-0.866025403784439));
#53215=DIRECTION('center_axis',(0.,0.,1.));
#53216=DIRECTION('ref_axis',(1.,0.,0.));
#53217=DIRECTION('center_axis',(0.,0.,-1.));
#53218=DIRECTION('ref_axis',(0.,1.,0.));
#53219=DIRECTION('center_axis',(0.,0.,1.));
#53220=DIRECTION('ref_axis',(1.,0.,0.));
#53221=DIRECTION('',(0.,-1.,0.));
#53222=DIRECTION('center_axis',(0.,0.,1.));
#53223=DIRECTION('ref_axis',(0.,1.,0.));
#53224=DIRECTION('center_axis',(0.,0.,-1.));
#53225=DIRECTION('ref_axis',(-1.,0.,0.));
#53226=DIRECTION('center_axis',(0.,0.,-1.));
#53227=DIRECTION('ref_axis',(0.,-1.,0.));
#53228=DIRECTION('',(0.,1.,0.));
#53229=DIRECTION('center_axis',(-1.,0.,0.));
#53230=DIRECTION('ref_axis',(0.,-1.,0.));
#53231=DIRECTION('center_axis',(-1.,0.,0.));
#53232=DIRECTION('ref_axis',(0.,0.,-1.));
#53233=DIRECTION('center_axis',(-1.,0.,0.));
#53234=DIRECTION('ref_axis',(0.,0.,-1.));
#53235=DIRECTION('center_axis',(-1.,0.,0.));
#53236=DIRECTION('ref_axis',(0.,0.,-1.));
#53237=DIRECTION('center_axis',(-1.,0.,0.));
#53238=DIRECTION('ref_axis',(0.,0.,-1.));
#53239=DIRECTION('center_axis',(-1.,0.,0.));
#53240=DIRECTION('ref_axis',(0.,0.,-1.));
#53241=DIRECTION('center_axis',(-1.,0.,0.));
#53242=DIRECTION('ref_axis',(0.,0.,-1.));
#53243=DIRECTION('center_axis',(1.,0.,0.));
#53244=DIRECTION('ref_axis',(0.,0.,-1.));
#53245=DIRECTION('center_axis',(1.,0.,0.));
#53246=DIRECTION('ref_axis',(0.,0.,-1.));
#53247=DIRECTION('center_axis',(1.,0.,0.));
#53248=DIRECTION('ref_axis',(0.,0.,-1.));
#53249=DIRECTION('center_axis',(0.,0.,1.));
#53250=DIRECTION('ref_axis',(1.,0.,0.));
#53251=DIRECTION('center_axis',(-1.,0.,0.));
#53252=DIRECTION('ref_axis',(0.,0.,1.));
#53253=DIRECTION('center_axis',(1.,0.,0.));
#53254=DIRECTION('ref_axis',(0.,0.,-1.));
#53255=DIRECTION('center_axis',(1.,0.,0.));
#53256=DIRECTION('ref_axis',(0.,0.,-1.));
#53257=DIRECTION('center_axis',(0.,0.,1.));
#53258=DIRECTION('ref_axis',(1.,0.,0.));
#53259=DIRECTION('center_axis',(1.22464679914735E-16,-1.,0.));
#53260=DIRECTION('ref_axis',(-1.,-1.22464679914735E-16,0.));
#53261=DIRECTION('center_axis',(1.22464679914735E-16,-1.,0.));
#53262=DIRECTION('ref_axis',(-1.,-1.22464679914735E-16,0.));
#81058=CARTESIAN_POINT('',(0.,0.,0.));
#81059=CARTESIAN_POINT('Origin',(150.,22.459292143521,-15.900635094611));
#81060=CARTESIAN_POINT('',(158.1,22.6393946667659,-16.2125818154424));
#81061=CARTESIAN_POINT('',(141.9,22.6393946667659,-16.2125818154424));
#81062=CARTESIAN_POINT('Origin',(150.,9.95929214352105,5.75));
#81063=CARTESIAN_POINT('',(158.1,19.9185842870421,-11.5));
#81064=CARTESIAN_POINT('',(158.1,17.459292143521,-7.24038105676659));
#81065=CARTESIAN_POINT('',(156.855654600401,19.9185842870421,-11.5));
#81066=CARTESIAN_POINT('',(150.,19.9185842870421,-11.5));
#81067=CARTESIAN_POINT('',(143.144345399599,19.9185842870421,-11.5));
#81068=CARTESIAN_POINT('Origin',(150.,9.95929214352105,5.75));
#81069=CARTESIAN_POINT('',(141.9,19.9185842870421,-11.5));
#81070=CARTESIAN_POINT('',(150.,19.9185842870421,-11.5));
#81071=CARTESIAN_POINT('',(141.9,27.459292143521,-24.5608891324554));
#81072=CARTESIAN_POINT('Origin',(150.,2.54070785647893,-27.400635094611));
#81073=CARTESIAN_POINT('',(141.9,2.72081037972379,-27.7125818154424));
#81074=CARTESIAN_POINT('',(158.1,2.72081037972379,-27.7125818154424));
#81075=CARTESIAN_POINT('Origin',(150.,-9.95929214352105,-5.74999999999998));
#81076=CARTESIAN_POINT('',(141.9,-1.4432899320127E-14,-23.));
#81077=CARTESIAN_POINT('',(141.9,7.54070785647893,-36.0608891324554));
#81078=CARTESIAN_POINT('',(143.144345399599,-1.4432899320127E-14,-23.));
#81079=CARTESIAN_POINT('',(150.,-1.4432899320127E-14,-23.));
#81080=CARTESIAN_POINT('',(156.855654600401,-1.4432899320127E-14,-23.));
#81081=CARTESIAN_POINT('Origin',(150.,-9.95929214352105,-5.74999999999998));
#81082=CARTESIAN_POINT('',(158.1,-1.55431223447522E-14,-23.));
#81083=CARTESIAN_POINT('',(150.,-1.4432899320127E-14,-23.));
#81084=CARTESIAN_POINT('',(158.1,-2.45929214352106,-18.7403810567666));
#81085=CARTESIAN_POINT('Origin',(158.1,15.,0.));
#81086=CARTESIAN_POINT('',(158.1,-2.72081037972383,-27.7125818154424));
#81087=CARTESIAN_POINT('',(158.1,2.45929214352104,-18.7403810567666));
#81088=CARTESIAN_POINT('',(158.1,-22.6393946667659,-16.2125818154424));
#81089=CARTESIAN_POINT('Origin',(158.1,-1.77635683940025E-14,0.));
#81090=CARTESIAN_POINT('',(158.1,-19.9185842870421,-11.5));
#81091=CARTESIAN_POINT('',(158.1,-17.459292143521,-7.24038105676657));
#81092=CARTESIAN_POINT('',(158.1,-25.3602050464897,-11.5));
#81093=CARTESIAN_POINT('',(158.1,-15.,-11.5));
#81094=CARTESIAN_POINT('',(158.1,-25.3602050464897,11.5));
#81095=CARTESIAN_POINT('Origin',(158.1,-1.77635683940025E-14,0.));
#81096=CARTESIAN_POINT('',(158.1,-19.9185842870421,11.5));
#81097=CARTESIAN_POINT('',(158.1,-15.,11.5));
#81098=CARTESIAN_POINT('',(158.1,-22.6393946667659,16.2125818154424));
#81099=CARTESIAN_POINT('',(158.1,-17.459292143521,7.24038105676658));
#81100=CARTESIAN_POINT('',(158.1,-2.7208103797238,27.7125818154424));
#81101=CARTESIAN_POINT('Origin',(158.1,-1.77635683940025E-14,0.));
#81102=CARTESIAN_POINT('',(158.1,4.71844785465692E-15,23.));
#81103=CARTESIAN_POINT('',(158.1,2.45929214352105,18.7403810567666));
#81104=CARTESIAN_POINT('',(158.1,2.72081037972381,27.7125818154424));
#81105=CARTESIAN_POINT('',(158.1,-2.45929214352104,18.7403810567666));
#81106=CARTESIAN_POINT('',(158.1,22.6393946667659,16.2125818154424));
#81107=CARTESIAN_POINT('Origin',(158.1,-1.77635683940025E-14,0.));
#81108=CARTESIAN_POINT('',(158.1,19.9185842870421,11.5));
#81109=CARTESIAN_POINT('',(158.1,17.459292143521,7.24038105676658));
#81110=CARTESIAN_POINT('',(158.1,25.3602050464897,11.5));
#81111=CARTESIAN_POINT('',(158.1,15.,11.5));
#81112=CARTESIAN_POINT('',(158.1,25.3602050464897,-11.5));
#81113=CARTESIAN_POINT('Origin',(158.1,-1.77635683940025E-14,0.));
#81114=CARTESIAN_POINT('',(158.1,15.,-11.5));
#81115=CARTESIAN_POINT('Origin',(158.1,-1.77635683940025E-14,0.));
#81116=CARTESIAN_POINT('',(158.1,0.236381056814519,-22.5905759996504));
#81117=CARTESIAN_POINT('Origin',(158.1,-1.77635683940025E-14,0.));
#81118=CARTESIAN_POINT('Origin',(150.,-2.54070785647897,-27.400635094611));
#81119=CARTESIAN_POINT('Origin',(150.,9.95929214352104,-5.75000000000001));
#81120=CARTESIAN_POINT('',(141.9,-2.72081037972383,-27.7125818154424));
#81121=CARTESIAN_POINT('',(141.9,-7.54070785647897,-36.0608891324554));
#81122=CARTESIAN_POINT('Origin',(150.,9.95929214352104,-5.75000000000001));
#81123=CARTESIAN_POINT('Origin',(150.,-1.77635683940025E-14,0.));
#81124=CARTESIAN_POINT('',(141.9,19.6822032302275,-11.0905759996504));
#81125=CARTESIAN_POINT('Origin',(141.9,-1.77635683940025E-14,0.));
#81126=CARTESIAN_POINT('',(140.,21.8174242292714,0.));
#81127=CARTESIAN_POINT('Origin',(140.,0.,0.));
#81128=CARTESIAN_POINT('Origin',(150.,-1.77635683940025E-14,0.));
#81129=CARTESIAN_POINT('',(150.,-1.77635683940025E-14,-24.));
#81130=CARTESIAN_POINT('Origin',(150.,-1.77635683940025E-14,0.));
#81131=CARTESIAN_POINT('Origin',(150.,-1.77635683940025E-14,0.));
#81132=CARTESIAN_POINT('Origin',(150.,-1.77635683940025E-14,-11.5));
#81133=CARTESIAN_POINT('Origin',(150.,-22.4592921435211,-15.900635094611));
#81134=CARTESIAN_POINT('',(156.855654600401,-19.9185842870421,-11.5));
#81135=CARTESIAN_POINT('',(150.,-19.9185842870421,-11.5));
#81136=CARTESIAN_POINT('',(141.9,-22.6393946667659,-16.2125818154424));
#81137=CARTESIAN_POINT('Origin',(150.,-9.95929214352105,5.75));
#81138=CARTESIAN_POINT('',(141.9,-19.9185842870421,-11.5));
#81139=CARTESIAN_POINT('',(141.9,-27.4592921435211,-24.5608891324553));
#81140=CARTESIAN_POINT('',(143.144345399599,-19.9185842870421,-11.5));
#81141=CARTESIAN_POINT('',(150.,-19.9185842870421,-11.5));
#81142=CARTESIAN_POINT('Origin',(150.,-9.95929214352105,5.75));
#81143=CARTESIAN_POINT('Origin',(150.,-1.77635683940025E-14,0.));
#81144=CARTESIAN_POINT('Origin',(150.,-1.9171912213022E-14,-11.5));
#81145=CARTESIAN_POINT('Origin',(150.,-25.,-11.5));
#81146=CARTESIAN_POINT('',(141.9,-25.3602050464897,-11.5));
#81147=CARTESIAN_POINT('',(141.9,-35.,-11.5));
#81148=CARTESIAN_POINT('Origin',(150.,-1.9171912213022E-14,-11.5));
#81149=CARTESIAN_POINT('Origin',(150.,-25.,11.5));
#81150=CARTESIAN_POINT('',(156.855654600401,-19.9185842870421,11.5));
#81151=CARTESIAN_POINT('',(150.,-19.9185842870421,11.5));
#81152=CARTESIAN_POINT('',(141.9,-25.3602050464897,11.5));
#81153=CARTESIAN_POINT('Origin',(150.,-1.63552245749831E-14,11.5));
#81154=CARTESIAN_POINT('',(141.9,-19.9185842870421,11.5));
#81155=CARTESIAN_POINT('',(141.9,-35.,11.5));
#81156=CARTESIAN_POINT('',(143.144345399599,-19.9185842870421,11.5));
#81157=CARTESIAN_POINT('',(150.,-19.9185842870421,11.5));
#81158=CARTESIAN_POINT('Origin',(150.,-1.63552245749831E-14,11.5));
#81159=CARTESIAN_POINT('Origin',(150.,-1.77635683940025E-14,0.));
#81160=CARTESIAN_POINT('Origin',(150.,-9.95929214352105,-5.74999999999999));
#81161=CARTESIAN_POINT('Origin',(150.,-22.459292143521,15.900635094611));
#81162=CARTESIAN_POINT('',(141.9,-22.6393946667659,16.2125818154424));
#81163=CARTESIAN_POINT('',(141.9,-27.459292143521,24.5608891324554));
#81164=CARTESIAN_POINT('Origin',(150.,-9.95929214352105,-5.74999999999999));
#81165=CARTESIAN_POINT('Origin',(150.,-2.54070785647895,27.400635094611));
#81166=CARTESIAN_POINT('',(156.855654600401,5.55111512312578E-15,23.));
#81167=CARTESIAN_POINT('',(150.,4.44089209850063E-15,23.));
#81168=CARTESIAN_POINT('',(141.9,-2.7208103797238,27.7125818154424));
#81169=CARTESIAN_POINT('Origin',(150.,9.95929214352105,5.75000000000001));
#81170=CARTESIAN_POINT('',(141.9,4.44089209850063E-15,23.));
#81171=CARTESIAN_POINT('',(141.9,-7.54070785647895,36.0608891324554));
#81172=CARTESIAN_POINT('',(143.144345399599,5.55111512312578E-15,23.));
#81173=CARTESIAN_POINT('',(150.,4.44089209850063E-15,23.));
#81174=CARTESIAN_POINT('Origin',(150.,9.95929214352105,5.75000000000001));
#81175=CARTESIAN_POINT('Origin',(150.,-1.77635683940025E-14,0.));
#81176=CARTESIAN_POINT('',(150.,-1.77635683940025E-14,24.));
#81177=CARTESIAN_POINT('Origin',(150.,-1.77635683940025E-14,0.));
#81178=CARTESIAN_POINT('Origin',(150.,-9.95929214352105,5.74999999999999));
#81179=CARTESIAN_POINT('Origin',(150.,2.54070785647896,27.400635094611));
#81180=CARTESIAN_POINT('',(141.9,2.72081037972381,27.7125818154424));
#81181=CARTESIAN_POINT('',(141.9,7.54070785647896,36.0608891324554));
#81182=CARTESIAN_POINT('Origin',(150.,-9.95929214352105,5.74999999999999));
#81183=CARTESIAN_POINT('Origin',(150.,22.459292143521,15.900635094611));
#81184=CARTESIAN_POINT('',(156.855654600401,19.9185842870421,11.5));
#81185=CARTESIAN_POINT('',(150.,19.9185842870421,11.5));
#81186=CARTESIAN_POINT('',(141.9,22.6393946667659,16.2125818154424));
#81187=CARTESIAN_POINT('Origin',(150.,9.95929214352104,-5.75000000000001));
#81188=CARTESIAN_POINT('',(141.9,19.9185842870421,11.5));
#81189=CARTESIAN_POINT('',(141.9,27.459292143521,24.5608891324554));
#81190=CARTESIAN_POINT('',(143.144345399599,19.9185842870421,11.5));
#81191=CARTESIAN_POINT('',(150.,19.9185842870421,11.5));
#81192=CARTESIAN_POINT('Origin',(150.,9.95929214352104,-5.75000000000001));
#81193=CARTESIAN_POINT('Origin',(150.,-1.77635683940025E-14,0.));
#81194=CARTESIAN_POINT('Origin',(150.,-1.77635683940025E-14,11.5));
#81195=CARTESIAN_POINT('Origin',(150.,25.,11.5));
#81196=CARTESIAN_POINT('',(141.9,25.3602050464897,11.5));
#81197=CARTESIAN_POINT('',(141.9,35.,11.5));
#81198=CARTESIAN_POINT('Origin',(150.,-1.77635683940025E-14,11.5));
#81199=CARTESIAN_POINT('Origin',(150.,25.,-11.5));
#81200=CARTESIAN_POINT('',(141.9,25.3602050464897,-11.5));
#81201=CARTESIAN_POINT('Origin',(150.,-1.77635683940025E-14,-11.5));
#81202=CARTESIAN_POINT('',(141.9,35.,-11.5));
#81203=CARTESIAN_POINT('Origin',(141.9,35.,0.));
#81204=CARTESIAN_POINT('Origin',(141.9,-1.77635683940025E-14,0.));
#81205=CARTESIAN_POINT('Origin',(141.9,-1.77635683940025E-14,0.));
#81206=CARTESIAN_POINT('Origin',(141.9,-1.77635683940025E-14,0.));
#81207=CARTESIAN_POINT('Origin',(141.9,-1.77635683940025E-14,0.));
#81208=CARTESIAN_POINT('Origin',(141.9,-1.77635683940025E-14,0.));
#81209=CARTESIAN_POINT('Origin',(141.9,-1.77635683940025E-14,0.));
#81210=CARTESIAN_POINT('Origin',(160.,21.8174242292714,0.));
#81211=CARTESIAN_POINT('',(160.,27.2213151776324,0.));
#81212=CARTESIAN_POINT('Origin',(160.,0.,0.));
#81213=CARTESIAN_POINT('',(160.,21.8174242292714,0.));
#81214=CARTESIAN_POINT('Origin',(160.,0.,0.));
#81215=CARTESIAN_POINT('Origin',(150.,-1.77635683940025E-14,0.));
#81216=CARTESIAN_POINT('Origin',(140.,27.2213151776324,0.));
#81217=CARTESIAN_POINT('',(140.,-1.89882151931499E-14,-27.2213151776324));
#81218=CARTESIAN_POINT('',(140.,-1.89882151931499E-14,27.2213151776324));
#81219=CARTESIAN_POINT('Origin',(140.,0.,0.));
#81220=CARTESIAN_POINT('Origin',(140.,0.,0.));
#81221=CARTESIAN_POINT('Origin',(150.,-1.77635683940025E-14,0.));
#81222=CARTESIAN_POINT('',(150.,-1.77635683940025E-14,29.));
#81223=CARTESIAN_POINT('Origin',(150.,-1.77635683940025E-14,0.));
#81224=CARTESIAN_POINT('',(150.,-1.77635683940025E-14,-29.));
#81225=CARTESIAN_POINT('Origin',(150.,-1.77635683940025E-14,0.));
#90342=UNCERTAINTY_MEASURE_WITH_UNIT(LENGTH_MEASURE(0.01),#90375,
'DISTANCE_ACCURACY_VALUE',
'Maximum model space distance between geometric entities at asserted c
onnectivities');
#90355=UNCERTAINTY_MEASURE_WITH_UNIT(LENGTH_MEASURE(0.01),#90375,
'DISTANCE_ACCURACY_VALUE',
'Maximum model space distance between geometric entities at asserted c
onnectivities');
#90361=(
GEOMETRIC_REPRESENTATION_CONTEXT(3)
GLOBAL_UNCERTAINTY_ASSIGNED_CONTEXT((#90342))
GLOBAL_UNIT_ASSIGNED_CONTEXT((#90375,#90377,#90378))
REPRESENTATION_CONTEXT('','3D')
);
#90374=(
GEOMETRIC_REPRESENTATION_CONTEXT(3)
GLOBAL_UNCERTAINTY_ASSIGNED_CONTEXT((#90355))
GLOBAL_UNIT_ASSIGNED_CONTEXT((#90375,#90377,#90378))
REPRESENTATION_CONTEXT('','3D')
);
#90375=(
LENGTH_UNIT()
NAMED_UNIT(*)
SI_UNIT(.MILLI.,.METRE.)
);
#90377=(
NAMED_UNIT(*)
PLANE_ANGLE_UNIT()
SI_UNIT($,.RADIAN.)
);
#90378=(
NAMED_UNIT(*)
SI_UNIT($,.STERADIAN.)
SOLID_ANGLE_UNIT()
);
#90384=SHAPE_DEFINITION_REPRESENTATION(#90402,#90445);
#90402=PRODUCT_DEFINITION_SHAPE('',$,#90464);
#90445=SHAPE_REPRESENTATION('',(#43719),#90361);
#90458=PRODUCT_DEFINITION_CONTEXT('part definition',#90514,'design');
#90464=PRODUCT_DEFINITION('2026-10-11-12-53-10-149','05_Ball_Cage',#90482,
#90458);
#90482=PRODUCT_DEFINITION_FORMATION('',$,#90521);
#90514=APPLICATION_CONTEXT(
'Core Data for Automotive Mechanical Design Process');
#90515=PRODUCT_CONTEXT('part definition',#90514,'mechanical');
#90521=PRODUCT('2026-10-11-12-53-10-149','05_Ball_Cage',$,(#90515));
#90695=COLOUR_RGB('Off White',0.89,0.88,0.83);
#90696=FILL_AREA_STYLE_COLOUR('',#90695);
#90697=FILL_AREA_STYLE('',(#90696));
#90698=SURFACE_STYLE_FILL_AREA(#90697);
#90699=SURFACE_SIDE_STYLE('',(#90698));
#90700=SURFACE_STYLE_USAGE(.BOTH.,#90699);
#90701=PRESENTATION_STYLE_ASSIGNMENT((#90700));
ENDSEC;
END-ISO-10303-21;
